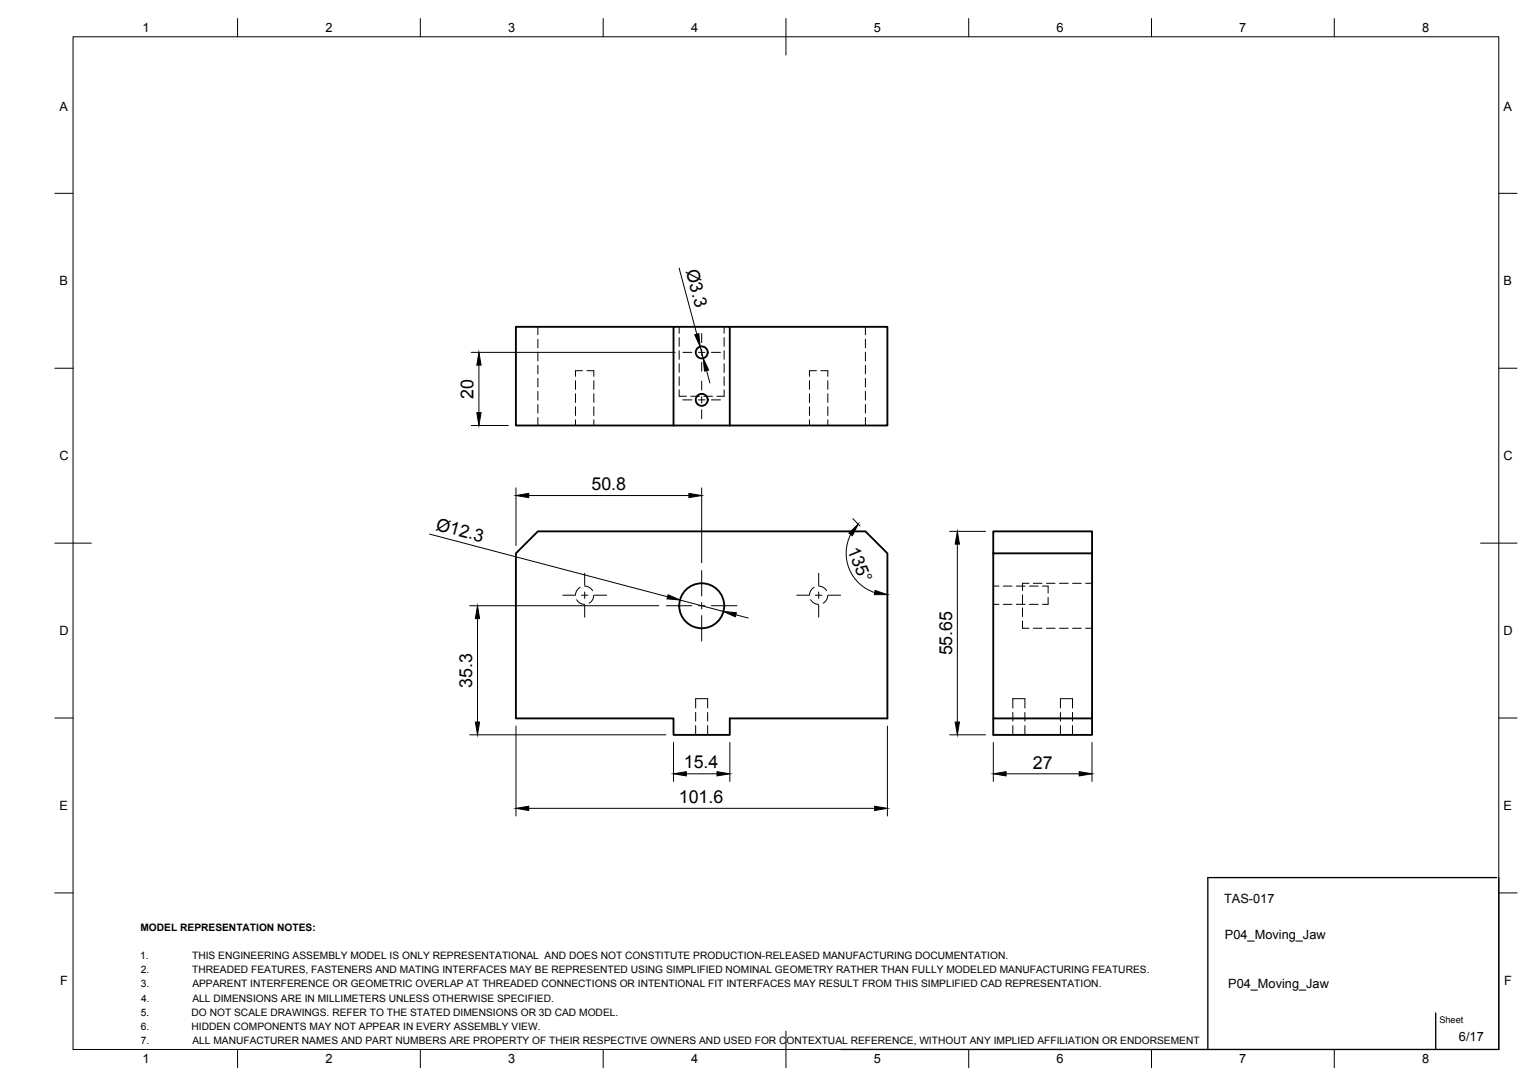
ISO-10303-21;
HEADER;
/* Generated by software containing ST-Developer
 * from STEP Tools, Inc. (www.steptools.com) 
 */

FILE_DESCRIPTION(
/* description */ ('STEP AP203'),
/* implementation_level */ '2;1');

FILE_NAME(
/* name */ 'P04_Moving_Jaw.step',
/* time_stamp */ '2026-11-15T15:04:01-08:00',
/* author */ (''),
/* organization */ (''),
/* preprocessor_version */ 'ST-DEVELOPER v20.2',
/* originating_system */ 'Autodesk Translation Framework v15.17.0.0',
/* authorisation */ '');

FILE_SCHEMA (('AUTOMOTIVE_DESIGN { 1 0 10303 214 3 1 1 }'));
ENDSEC;

DATA;
#10=MECHANICAL_DESIGN_GEOMETRIC_PRESENTATION_REPRESENTATION('',(#283,#284,#285),#16598);
#207=SHAPE_REPRESENTATION_RELATIONSHIP('SRR','None',#16701,#231);
#231=ADVANCED_BREP_SHAPE_REPRESENTATION('',(#255),#16577);
#255=MANIFOLD_SOLID_BREP('Body1',#9790);
#283=STYLED_ITEM('',(#16828),#9385);
#284=STYLED_ITEM('',(#16828),#9386);
#285=STYLED_ITEM('',(#16831),#255);
#331=FACE_BOUND('',#1644,.T.);
#332=FACE_BOUND('',#1645,.T.);
#333=FACE_BOUND('',#1647,.T.);
#334=FACE_BOUND('',#1651,.T.);
#335=FACE_BOUND('',#1652,.T.);
#558=PLANE('',#10282);
#559=PLANE('',#10283);
#560=PLANE('',#10284);
#561=PLANE('',#10285);
#562=PLANE('',#10286);
#563=PLANE('',#10287);
#564=PLANE('',#10288);
#565=PLANE('',#10289);
#566=PLANE('',#10290);
#567=PLANE('',#10291);
#568=PLANE('',#10292);
#569=PLANE('',#10293);
#570=PLANE('',#10294);
#571=PLANE('',#10295);
#572=PLANE('',#10296);
#573=PLANE('',#10297);
#574=PLANE('',#10298);
#1055=FACE_OUTER_BOUND('',#1631,.T.);
#1056=FACE_OUTER_BOUND('',#1632,.T.);
#1057=FACE_OUTER_BOUND('',#1633,.T.);
#1058=FACE_OUTER_BOUND('',#1634,.T.);
#1059=FACE_OUTER_BOUND('',#1635,.T.);
#1060=FACE_OUTER_BOUND('',#1636,.T.);
#1061=FACE_OUTER_BOUND('',#1637,.T.);
#1062=FACE_OUTER_BOUND('',#1638,.T.);
#1063=FACE_OUTER_BOUND('',#1639,.T.);
#1064=FACE_OUTER_BOUND('',#1640,.T.);
#1065=FACE_OUTER_BOUND('',#1641,.T.);
#1066=FACE_OUTER_BOUND('',#1642,.T.);
#1067=FACE_OUTER_BOUND('',#1643,.T.);
#1068=FACE_OUTER_BOUND('',#1646,.T.);
#1069=FACE_OUTER_BOUND('',#1648,.T.);
#1070=FACE_OUTER_BOUND('',#1649,.T.);
#1071=FACE_OUTER_BOUND('',#1650,.T.);
#1072=FACE_OUTER_BOUND('',#1653,.T.);
#1073=FACE_OUTER_BOUND('',#1654,.T.);
#1074=FACE_OUTER_BOUND('',#1655,.T.);
#1075=FACE_OUTER_BOUND('',#1656,.T.);
#1076=FACE_OUTER_BOUND('',#1657,.T.);
#1631=EDGE_LOOP('',(#7371,#7372,#7373,#7374));
#1632=EDGE_LOOP('',(#7375,#7376,#7377,#7378));
#1633=EDGE_LOOP('',(#7379,#7380,#7381,#7382));
#1634=EDGE_LOOP('',(#7383,#7384,#7385,#7386));
#1635=EDGE_LOOP('',(#7387,#7388,#7389,#7390));
#1636=EDGE_LOOP('',(#7391,#7392,#7393,#7394));
#1637=EDGE_LOOP('',(#7395,#7396,#7397,#7398));
#1638=EDGE_LOOP('',(#7399,#7400,#7401,#7402));
#1639=EDGE_LOOP('',(#7403,#7404,#7405,#7406));
#1640=EDGE_LOOP('',(#7407,#7408,#7409,#7410));
#1641=EDGE_LOOP('',(#7411,#7412,#7413,#7414));
#1642=EDGE_LOOP('',(#7415,#7416,#7417,#7418));
#1643=EDGE_LOOP('',(#7419,#7420,#7421,#7422,#7423,#7424,#7425,#7426,#7427,
#7428));
#1644=EDGE_LOOP('',(#7429));
#1645=EDGE_LOOP('',(#7430));
#1646=EDGE_LOOP('',(#7431,#7432,#7433,#7434,#7435,#7436,#7437,#7438,#7439,
#7440));
#1647=EDGE_LOOP('',(#7441));
#1648=EDGE_LOOP('',(#7442,#7443,#7444,#7445));
#1649=EDGE_LOOP('',(#7446,#7447,#7448,#7449));
#1650=EDGE_LOOP('',(#7450,#7451,#7452,#7453));
#1651=EDGE_LOOP('',(#7454));
#1652=EDGE_LOOP('',(#7455));
#1653=EDGE_LOOP('',(#7456));
#1654=EDGE_LOOP('',(#7457));
#1655=EDGE_LOOP('',(#7458));
#1656=EDGE_LOOP('',(#7459));
#1657=EDGE_LOOP('',(#7460));
#2481=LINE('',#14478,#3529);
#2482=LINE('',#14484,#3530);
#2483=LINE('',#14490,#3531);
#2484=LINE('',#14496,#3532);
#2485=LINE('',#14502,#3533);
#2486=LINE('',#14507,#3534);
#2487=LINE('',#14509,#3535);
#2488=LINE('',#14511,#3536);
#2489=LINE('',#14512,#3537);
#2490=LINE('',#14516,#3538);
#2491=LINE('',#14518,#3539);
#2492=LINE('',#14520,#3540);
#2493=LINE('',#14521,#3541);
#2494=LINE('',#14524,#3542);
#2495=LINE('',#14526,#3543);
#2496=LINE('',#14527,#3544);
#2497=LINE('',#14530,#3545);
#2498=LINE('',#14532,#3546);
#2499=LINE('',#14533,#3547);
#2500=LINE('',#14536,#3548);
#2501=LINE('',#14538,#3549);
#2502=LINE('',#14539,#3550);
#2503=LINE('',#14542,#3551);
#2504=LINE('',#14544,#3552);
#2505=LINE('',#14545,#3553);
#2506=LINE('',#14547,#3554);
#2507=LINE('',#14548,#3555);
#2508=LINE('',#14551,#3556);
#2509=LINE('',#14553,#3557);
#2510=LINE('',#14554,#3558);
#2511=LINE('',#14557,#3559);
#2512=LINE('',#14559,#3560);
#2513=LINE('',#14560,#3561);
#2514=LINE('',#14562,#3562);
#2515=LINE('',#14564,#3563);
#3529=VECTOR('',#11659,1.65);
#3530=VECTOR('',#11666,1.65);
#3531=VECTOR('',#11673,2.5);
#3532=VECTOR('',#11680,2.5);
#3533=VECTOR('',#11687,6.15);
#3534=VECTOR('',#11692,1000.);
#3535=VECTOR('',#11693,1000.);
#3536=VECTOR('',#11694,1000.);
#3537=VECTOR('',#11695,1000.);
#3538=VECTOR('',#11698,1000.);
#3539=VECTOR('',#11699,1000.);
#3540=VECTOR('',#11700,1000.);
#3541=VECTOR('',#11701,1000.);
#3542=VECTOR('',#11704,1000.);
#3543=VECTOR('',#11705,1000.);
#3544=VECTOR('',#11706,1000.);
#3545=VECTOR('',#11709,1000.);
#3546=VECTOR('',#11710,1000.);
#3547=VECTOR('',#11711,1000.);
#3548=VECTOR('',#11714,1000.);
#3549=VECTOR('',#11715,1000.);
#3550=VECTOR('',#11716,1000.);
#3551=VECTOR('',#11719,1000.);
#3552=VECTOR('',#11720,1000.);
#3553=VECTOR('',#11721,1000.);
#3554=VECTOR('',#11724,1000.);
#3555=VECTOR('',#11725,1000.);
#3556=VECTOR('',#11728,1000.);
#3557=VECTOR('',#11729,1000.);
#3558=VECTOR('',#11730,1000.);
#3559=VECTOR('',#11733,1000.);
#3560=VECTOR('',#11734,1000.);
#3561=VECTOR('',#11735,1000.);
#3562=VECTOR('',#11738,1000.);
#3563=VECTOR('',#11741,1000.);
#4265=CIRCLE('',#10268,1.65);
#4266=CIRCLE('',#10269,1.65);
#4267=CIRCLE('',#10271,1.65);
#4268=CIRCLE('',#10272,1.65);
#4269=CIRCLE('',#10274,2.5);
#4270=CIRCLE('',#10275,2.5);
#4271=CIRCLE('',#10277,2.5);
#4272=CIRCLE('',#10278,2.5);
#4273=CIRCLE('',#10280,6.15);
#4274=CIRCLE('',#10281,6.15);
#4713=VERTEX_POINT('',#14475);
#4714=VERTEX_POINT('',#14477);
#4715=VERTEX_POINT('',#14481);
#4716=VERTEX_POINT('',#14483);
#4717=VERTEX_POINT('',#14487);
#4718=VERTEX_POINT('',#14489);
#4719=VERTEX_POINT('',#14493);
#4720=VERTEX_POINT('',#14495);
#4721=VERTEX_POINT('',#14499);
#4722=VERTEX_POINT('',#14501);
#4723=VERTEX_POINT('',#14505);
#4724=VERTEX_POINT('',#14506);
#4725=VERTEX_POINT('',#14508);
#4726=VERTEX_POINT('',#14510);
#4727=VERTEX_POINT('',#14514);
#4728=VERTEX_POINT('',#14515);
#4729=VERTEX_POINT('',#14517);
#4730=VERTEX_POINT('',#14519);
#4731=VERTEX_POINT('',#14523);
#4732=VERTEX_POINT('',#14525);
#4733=VERTEX_POINT('',#14529);
#4734=VERTEX_POINT('',#14531);
#4735=VERTEX_POINT('',#14535);
#4736=VERTEX_POINT('',#14537);
#4737=VERTEX_POINT('',#14541);
#4738=VERTEX_POINT('',#14543);
#4739=VERTEX_POINT('',#14550);
#4740=VERTEX_POINT('',#14552);
#4741=VERTEX_POINT('',#14556);
#4742=VERTEX_POINT('',#14558);
#5698=EDGE_CURVE('',#4713,#4713,#4265,.T.);
#5699=EDGE_CURVE('',#4713,#4714,#2481,.T.);
#5700=EDGE_CURVE('',#4714,#4714,#4266,.T.);
#5701=EDGE_CURVE('',#4715,#4715,#4267,.T.);
#5702=EDGE_CURVE('',#4715,#4716,#2482,.T.);
#5703=EDGE_CURVE('',#4716,#4716,#4268,.T.);
#5704=EDGE_CURVE('',#4717,#4717,#4269,.T.);
#5705=EDGE_CURVE('',#4717,#4718,#2483,.T.);
#5706=EDGE_CURVE('',#4718,#4718,#4270,.T.);
#5707=EDGE_CURVE('',#4719,#4719,#4271,.T.);
#5708=EDGE_CURVE('',#4719,#4720,#2484,.T.);
#5709=EDGE_CURVE('',#4720,#4720,#4272,.T.);
#5710=EDGE_CURVE('',#4721,#4721,#4273,.T.);
#5711=EDGE_CURVE('',#4721,#4722,#2485,.T.);
#5712=EDGE_CURVE('',#4722,#4722,#4274,.T.);
#5713=EDGE_CURVE('',#4723,#4724,#2486,.T.);
#5714=EDGE_CURVE('',#4725,#4723,#2487,.T.);
#5715=EDGE_CURVE('',#4725,#4726,#2488,.T.);
#5716=EDGE_CURVE('',#4726,#4724,#2489,.T.);
#5717=EDGE_CURVE('',#4727,#4728,#2490,.T.);
#5718=EDGE_CURVE('',#4727,#4729,#2491,.T.);
#5719=EDGE_CURVE('',#4730,#4729,#2492,.T.);
#5720=EDGE_CURVE('',#4728,#4730,#2493,.T.);
#5721=EDGE_CURVE('',#4729,#4731,#2494,.T.);
#5722=EDGE_CURVE('',#4732,#4731,#2495,.T.);
#5723=EDGE_CURVE('',#4730,#4732,#2496,.T.);
#5724=EDGE_CURVE('',#4731,#4733,#2497,.T.);
#5725=EDGE_CURVE('',#4734,#4733,#2498,.T.);
#5726=EDGE_CURVE('',#4732,#4734,#2499,.T.);
#5727=EDGE_CURVE('',#4733,#4735,#2500,.T.);
#5728=EDGE_CURVE('',#4736,#4735,#2501,.T.);
#5729=EDGE_CURVE('',#4734,#4736,#2502,.T.);
#5730=EDGE_CURVE('',#4735,#4737,#2503,.T.);
#5731=EDGE_CURVE('',#4738,#4737,#2504,.T.);
#5732=EDGE_CURVE('',#4736,#4738,#2505,.T.);
#5733=EDGE_CURVE('',#4737,#4726,#2506,.T.);
#5734=EDGE_CURVE('',#4738,#4725,#2507,.T.);
#5735=EDGE_CURVE('',#4723,#4739,#2508,.T.);
#5736=EDGE_CURVE('',#4739,#4740,#2509,.T.);
#5737=EDGE_CURVE('',#4728,#4740,#2510,.T.);
#5738=EDGE_CURVE('',#4727,#4741,#2511,.T.);
#5739=EDGE_CURVE('',#4741,#4742,#2512,.T.);
#5740=EDGE_CURVE('',#4724,#4742,#2513,.T.);
#5741=EDGE_CURVE('',#4742,#4739,#2514,.T.);
#5742=EDGE_CURVE('',#4740,#4741,#2515,.T.);
#7371=ORIENTED_EDGE('',*,*,#5698,.T.);
#7372=ORIENTED_EDGE('',*,*,#5699,.T.);
#7373=ORIENTED_EDGE('',*,*,#5700,.F.);
#7374=ORIENTED_EDGE('',*,*,#5699,.F.);
#7375=ORIENTED_EDGE('',*,*,#5701,.T.);
#7376=ORIENTED_EDGE('',*,*,#5702,.T.);
#7377=ORIENTED_EDGE('',*,*,#5703,.F.);
#7378=ORIENTED_EDGE('',*,*,#5702,.F.);
#7379=ORIENTED_EDGE('',*,*,#5704,.T.);
#7380=ORIENTED_EDGE('',*,*,#5705,.T.);
#7381=ORIENTED_EDGE('',*,*,#5706,.F.);
#7382=ORIENTED_EDGE('',*,*,#5705,.F.);
#7383=ORIENTED_EDGE('',*,*,#5707,.T.);
#7384=ORIENTED_EDGE('',*,*,#5708,.T.);
#7385=ORIENTED_EDGE('',*,*,#5709,.F.);
#7386=ORIENTED_EDGE('',*,*,#5708,.F.);
#7387=ORIENTED_EDGE('',*,*,#5710,.T.);
#7388=ORIENTED_EDGE('',*,*,#5711,.T.);
#7389=ORIENTED_EDGE('',*,*,#5712,.F.);
#7390=ORIENTED_EDGE('',*,*,#5711,.F.);
#7391=ORIENTED_EDGE('',*,*,#5713,.F.);
#7392=ORIENTED_EDGE('',*,*,#5714,.F.);
#7393=ORIENTED_EDGE('',*,*,#5715,.T.);
#7394=ORIENTED_EDGE('',*,*,#5716,.T.);
#7395=ORIENTED_EDGE('',*,*,#5717,.F.);
#7396=ORIENTED_EDGE('',*,*,#5718,.T.);
#7397=ORIENTED_EDGE('',*,*,#5719,.F.);
#7398=ORIENTED_EDGE('',*,*,#5720,.F.);
#7399=ORIENTED_EDGE('',*,*,#5721,.T.);
#7400=ORIENTED_EDGE('',*,*,#5722,.F.);
#7401=ORIENTED_EDGE('',*,*,#5723,.F.);
#7402=ORIENTED_EDGE('',*,*,#5719,.T.);
#7403=ORIENTED_EDGE('',*,*,#5724,.T.);
#7404=ORIENTED_EDGE('',*,*,#5725,.F.);
#7405=ORIENTED_EDGE('',*,*,#5726,.F.);
#7406=ORIENTED_EDGE('',*,*,#5722,.T.);
#7407=ORIENTED_EDGE('',*,*,#5727,.T.);
#7408=ORIENTED_EDGE('',*,*,#5728,.F.);
#7409=ORIENTED_EDGE('',*,*,#5729,.F.);
#7410=ORIENTED_EDGE('',*,*,#5725,.T.);
#7411=ORIENTED_EDGE('',*,*,#5730,.T.);
#7412=ORIENTED_EDGE('',*,*,#5731,.F.);
#7413=ORIENTED_EDGE('',*,*,#5732,.F.);
#7414=ORIENTED_EDGE('',*,*,#5728,.T.);
#7415=ORIENTED_EDGE('',*,*,#5733,.T.);
#7416=ORIENTED_EDGE('',*,*,#5715,.F.);
#7417=ORIENTED_EDGE('',*,*,#5734,.F.);
#7418=ORIENTED_EDGE('',*,*,#5731,.T.);
#7419=ORIENTED_EDGE('',*,*,#5714,.T.);
#7420=ORIENTED_EDGE('',*,*,#5735,.T.);
#7421=ORIENTED_EDGE('',*,*,#5736,.T.);
#7422=ORIENTED_EDGE('',*,*,#5737,.F.);
#7423=ORIENTED_EDGE('',*,*,#5720,.T.);
#7424=ORIENTED_EDGE('',*,*,#5723,.T.);
#7425=ORIENTED_EDGE('',*,*,#5726,.T.);
#7426=ORIENTED_EDGE('',*,*,#5729,.T.);
#7427=ORIENTED_EDGE('',*,*,#5732,.T.);
#7428=ORIENTED_EDGE('',*,*,#5734,.T.);
#7429=ORIENTED_EDGE('',*,*,#5704,.F.);
#7430=ORIENTED_EDGE('',*,*,#5707,.F.);
#7431=ORIENTED_EDGE('',*,*,#5718,.F.);
#7432=ORIENTED_EDGE('',*,*,#5738,.T.);
#7433=ORIENTED_EDGE('',*,*,#5739,.T.);
#7434=ORIENTED_EDGE('',*,*,#5740,.F.);
#7435=ORIENTED_EDGE('',*,*,#5716,.F.);
#7436=ORIENTED_EDGE('',*,*,#5733,.F.);
#7437=ORIENTED_EDGE('',*,*,#5730,.F.);
#7438=ORIENTED_EDGE('',*,*,#5727,.F.);
#7439=ORIENTED_EDGE('',*,*,#5724,.F.);
#7440=ORIENTED_EDGE('',*,*,#5721,.F.);
#7441=ORIENTED_EDGE('',*,*,#5712,.T.);
#7442=ORIENTED_EDGE('',*,*,#5735,.F.);
#7443=ORIENTED_EDGE('',*,*,#5713,.T.);
#7444=ORIENTED_EDGE('',*,*,#5740,.T.);
#7445=ORIENTED_EDGE('',*,*,#5741,.T.);
#7446=ORIENTED_EDGE('',*,*,#5738,.F.);
#7447=ORIENTED_EDGE('',*,*,#5717,.T.);
#7448=ORIENTED_EDGE('',*,*,#5737,.T.);
#7449=ORIENTED_EDGE('',*,*,#5742,.T.);
#7450=ORIENTED_EDGE('',*,*,#5741,.F.);
#7451=ORIENTED_EDGE('',*,*,#5739,.F.);
#7452=ORIENTED_EDGE('',*,*,#5742,.F.);
#7453=ORIENTED_EDGE('',*,*,#5736,.F.);
#7454=ORIENTED_EDGE('',*,*,#5700,.T.);
#7455=ORIENTED_EDGE('',*,*,#5703,.T.);
#7456=ORIENTED_EDGE('',*,*,#5710,.F.);
#7457=ORIENTED_EDGE('',*,*,#5709,.T.);
#7458=ORIENTED_EDGE('',*,*,#5706,.T.);
#7459=ORIENTED_EDGE('',*,*,#5701,.F.);
#7460=ORIENTED_EDGE('',*,*,#5698,.F.);
#9184=CYLINDRICAL_SURFACE('',#10267,1.65);
#9185=CYLINDRICAL_SURFACE('',#10270,1.65);
#9186=CYLINDRICAL_SURFACE('',#10273,2.5);
#9187=CYLINDRICAL_SURFACE('',#10276,2.5);
#9188=CYLINDRICAL_SURFACE('',#10279,6.15);
#9380=ADVANCED_FACE('',(#1055),#9184,.F.);
#9381=ADVANCED_FACE('',(#1056),#9185,.F.);
#9382=ADVANCED_FACE('',(#1057),#9186,.F.);
#9383=ADVANCED_FACE('',(#1058),#9187,.F.);
#9384=ADVANCED_FACE('',(#1059),#9188,.F.);
#9385=ADVANCED_FACE('',(#1060),#558,.F.);
#9386=ADVANCED_FACE('',(#1061),#559,.F.);
#9387=ADVANCED_FACE('',(#1062),#560,.F.);
#9388=ADVANCED_FACE('',(#1063),#561,.F.);
#9389=ADVANCED_FACE('',(#1064),#562,.F.);
#9390=ADVANCED_FACE('',(#1065),#563,.F.);
#9391=ADVANCED_FACE('',(#1066),#564,.F.);
#9392=ADVANCED_FACE('',(#1067,#331,#332),#565,.F.);
#9393=ADVANCED_FACE('',(#1068,#333),#566,.T.);
#9394=ADVANCED_FACE('',(#1069),#567,.F.);
#9395=ADVANCED_FACE('',(#1070),#568,.F.);
#9396=ADVANCED_FACE('',(#1071,#334,#335),#569,.T.);
#9397=ADVANCED_FACE('',(#1072),#570,.F.);
#9398=ADVANCED_FACE('',(#1073),#571,.T.);
#9399=ADVANCED_FACE('',(#1074),#572,.T.);
#9400=ADVANCED_FACE('',(#1075),#573,.F.);
#9401=ADVANCED_FACE('',(#1076),#574,.F.);
#9790=CLOSED_SHELL('',(#9380,#9381,#9382,#9383,#9384,#9385,#9386,#9387,
#9388,#9389,#9390,#9391,#9392,#9393,#9394,#9395,#9396,#9397,#9398,#9399,
#9400,#9401));
#10266=AXIS2_PLACEMENT_3D('',#14473,#11653,#11654);
#10267=AXIS2_PLACEMENT_3D('',#14474,#11655,#11656);
#10268=AXIS2_PLACEMENT_3D('',#14476,#11657,#11658);
#10269=AXIS2_PLACEMENT_3D('',#14479,#11660,#11661);
#10270=AXIS2_PLACEMENT_3D('',#14480,#11662,#11663);
#10271=AXIS2_PLACEMENT_3D('',#14482,#11664,#11665);
#10272=AXIS2_PLACEMENT_3D('',#14485,#11667,#11668);
#10273=AXIS2_PLACEMENT_3D('',#14486,#11669,#11670);
#10274=AXIS2_PLACEMENT_3D('',#14488,#11671,#11672);
#10275=AXIS2_PLACEMENT_3D('',#14491,#11674,#11675);
#10276=AXIS2_PLACEMENT_3D('',#14492,#11676,#11677);
#10277=AXIS2_PLACEMENT_3D('',#14494,#11678,#11679);
#10278=AXIS2_PLACEMENT_3D('',#14497,#11681,#11682);
#10279=AXIS2_PLACEMENT_3D('',#14498,#11683,#11684);
#10280=AXIS2_PLACEMENT_3D('',#14500,#11685,#11686);
#10281=AXIS2_PLACEMENT_3D('',#14503,#11688,#11689);
#10282=AXIS2_PLACEMENT_3D('',#14504,#11690,#11691);
#10283=AXIS2_PLACEMENT_3D('',#14513,#11696,#11697);
#10284=AXIS2_PLACEMENT_3D('',#14522,#11702,#11703);
#10285=AXIS2_PLACEMENT_3D('',#14528,#11707,#11708);
#10286=AXIS2_PLACEMENT_3D('',#14534,#11712,#11713);
#10287=AXIS2_PLACEMENT_3D('',#14540,#11717,#11718);
#10288=AXIS2_PLACEMENT_3D('',#14546,#11722,#11723);
#10289=AXIS2_PLACEMENT_3D('',#14549,#11726,#11727);
#10290=AXIS2_PLACEMENT_3D('',#14555,#11731,#11732);
#10291=AXIS2_PLACEMENT_3D('',#14561,#11736,#11737);
#10292=AXIS2_PLACEMENT_3D('',#14563,#11739,#11740);
#10293=AXIS2_PLACEMENT_3D('',#14565,#11742,#11743);
#10294=AXIS2_PLACEMENT_3D('',#14566,#11744,#11745);
#10295=AXIS2_PLACEMENT_3D('',#14567,#11746,#11747);
#10296=AXIS2_PLACEMENT_3D('',#14568,#11748,#11749);
#10297=AXIS2_PLACEMENT_3D('',#14569,#11750,#11751);
#10298=AXIS2_PLACEMENT_3D('',#14570,#11752,#11753);
#11653=DIRECTION('axis',(0.,0.,1.));
#11654=DIRECTION('refdir',(1.,0.,0.));
#11655=DIRECTION('center_axis',(0.,0.,-1.));
#11656=DIRECTION('ref_axis',(-1.,0.,0.));
#11657=DIRECTION('center_axis',(0.,0.,1.));
#11658=DIRECTION('ref_axis',(1.,0.,0.));
#11659=DIRECTION('',(0.,0.,-1.));
#11660=DIRECTION('center_axis',(0.,0.,1.));
#11661=DIRECTION('ref_axis',(-1.,0.,0.));
#11662=DIRECTION('center_axis',(0.,0.,-1.));
#11663=DIRECTION('ref_axis',(-1.,0.,0.));
#11664=DIRECTION('center_axis',(0.,0.,1.));
#11665=DIRECTION('ref_axis',(1.,0.,0.));
#11666=DIRECTION('',(0.,0.,-1.));
#11667=DIRECTION('center_axis',(0.,0.,1.));
#11668=DIRECTION('ref_axis',(-1.,0.,0.));
#11669=DIRECTION('center_axis',(0.,-1.,0.));
#11670=DIRECTION('ref_axis',(0.,0.,-1.));
#11671=DIRECTION('center_axis',(0.,1.,0.));
#11672=DIRECTION('ref_axis',(0.,0.,-1.));
#11673=DIRECTION('',(0.,-1.,0.));
#11674=DIRECTION('center_axis',(0.,1.,0.));
#11675=DIRECTION('ref_axis',(0.,0.,1.));
#11676=DIRECTION('center_axis',(0.,-1.,0.));
#11677=DIRECTION('ref_axis',(0.,0.,-1.));
#11678=DIRECTION('center_axis',(0.,1.,0.));
#11679=DIRECTION('ref_axis',(0.,0.,-1.));
#11680=DIRECTION('',(0.,-1.,0.));
#11681=DIRECTION('center_axis',(0.,1.,0.));
#11682=DIRECTION('ref_axis',(0.,0.,1.));
#11683=DIRECTION('center_axis',(0.,-1.,0.));
#11684=DIRECTION('ref_axis',(0.,0.,-1.));
#11685=DIRECTION('center_axis',(0.,1.,0.));
#11686=DIRECTION('ref_axis',(0.,0.,1.));
#11687=DIRECTION('',(0.,-1.,0.));
#11688=DIRECTION('center_axis',(0.,1.,0.));
#11689=DIRECTION('ref_axis',(0.,0.,-1.));
#11690=DIRECTION('center_axis',(0.,0.,1.));
#11691=DIRECTION('ref_axis',(1.,0.,0.));
#11692=DIRECTION('',(0.,-1.,0.));
#11693=DIRECTION('',(-1.,0.,0.));
#11694=DIRECTION('',(0.,-1.,0.));
#11695=DIRECTION('',(-1.,0.,0.));
#11696=DIRECTION('center_axis',(0.,0.,1.));
#11697=DIRECTION('ref_axis',(1.,0.,0.));
#11698=DIRECTION('',(0.,1.,0.));
#11699=DIRECTION('',(-1.,0.,0.));
#11700=DIRECTION('',(0.,-1.,0.));
#11701=DIRECTION('',(-1.,0.,0.));
#11702=DIRECTION('center_axis',(1.,0.,0.));
#11703=DIRECTION('ref_axis',(0.,0.,-1.));
#11704=DIRECTION('',(0.,0.,1.));
#11705=DIRECTION('',(0.,-1.,0.));
#11706=DIRECTION('',(0.,0.,1.));
#11707=DIRECTION('center_axis',(0.70710678118654,0.,-0.707106781186555));
#11708=DIRECTION('ref_axis',(-0.707106781186555,0.,-0.70710678118654));
#11709=DIRECTION('',(0.707106781186555,0.,0.70710678118654));
#11710=DIRECTION('',(0.,-1.,0.));
#11711=DIRECTION('',(0.707106781186555,0.,0.70710678118654));
#11712=DIRECTION('center_axis',(0.,0.,-1.));
#11713=DIRECTION('ref_axis',(-1.,0.,0.));
#11714=DIRECTION('',(1.,0.,0.));
#11715=DIRECTION('',(0.,-1.,0.));
#11716=DIRECTION('',(1.,0.,0.));
#11717=DIRECTION('center_axis',(-0.707106781186565,0.,-0.70710678118653));
#11718=DIRECTION('ref_axis',(-0.70710678118653,0.,0.707106781186565));
#11719=DIRECTION('',(0.70710678118653,0.,-0.707106781186565));
#11720=DIRECTION('',(0.,-1.,0.));
#11721=DIRECTION('',(0.70710678118653,0.,-0.707106781186565));
#11722=DIRECTION('center_axis',(-1.,0.,0.));
#11723=DIRECTION('ref_axis',(0.,0.,1.));
#11724=DIRECTION('',(0.,0.,-1.));
#11725=DIRECTION('',(0.,0.,-1.));
#11726=DIRECTION('center_axis',(0.,-1.,0.));
#11727=DIRECTION('ref_axis',(0.,0.,-1.));
#11728=DIRECTION('',(0.,0.,-1.));
#11729=DIRECTION('',(-1.,0.,0.));
#11730=DIRECTION('',(0.,0.,-1.));
#11731=DIRECTION('center_axis',(0.,-1.,0.));
#11732=DIRECTION('ref_axis',(0.,0.,-1.));
#11733=DIRECTION('',(0.,0.,-1.));
#11734=DIRECTION('',(1.,0.,0.));
#11735=DIRECTION('',(0.,0.,-1.));
#11736=DIRECTION('center_axis',(-1.,0.,0.));
#11737=DIRECTION('ref_axis',(0.,0.,1.));
#11738=DIRECTION('',(0.,1.,0.));
#11739=DIRECTION('center_axis',(1.,0.,0.));
#11740=DIRECTION('ref_axis',(0.,0.,-1.));
#11741=DIRECTION('',(0.,-1.,0.));
#11742=DIRECTION('center_axis',(0.,0.,-1.));
#11743=DIRECTION('ref_axis',(-1.,0.,0.));
#11744=DIRECTION('center_axis',(0.,1.,0.));
#11745=DIRECTION('ref_axis',(0.,0.,1.));
#11746=DIRECTION('center_axis',(0.,1.,0.));
#11747=DIRECTION('ref_axis',(0.,0.,1.));
#11748=DIRECTION('center_axis',(0.,1.,0.));
#11749=DIRECTION('ref_axis',(0.,0.,1.));
#11750=DIRECTION('center_axis',(0.,0.,1.));
#11751=DIRECTION('ref_axis',(1.,0.,0.));
#11752=DIRECTION('center_axis',(0.,0.,1.));
#11753=DIRECTION('ref_axis',(1.,0.,0.));
#14473=CARTESIAN_POINT('',(0.,0.,0.));
#14474=CARTESIAN_POINT('Origin',(0.,5.,87.6));
#14475=CARTESIAN_POINT('',(1.65,5.,87.6));
#14476=CARTESIAN_POINT('Origin',(0.,5.,87.6));
#14477=CARTESIAN_POINT('',(1.65,5.,77.7));
#14478=CARTESIAN_POINT('',(1.65,5.,87.6));
#14479=CARTESIAN_POINT('Origin',(0.,5.,77.7));
#14480=CARTESIAN_POINT('Origin',(0.,18.,87.6));
#14481=CARTESIAN_POINT('',(1.65,18.,87.6));
#14482=CARTESIAN_POINT('Origin',(0.,18.,87.6));
#14483=CARTESIAN_POINT('',(1.65,18.,77.7));
#14484=CARTESIAN_POINT('',(1.65,18.,87.6));
#14485=CARTESIAN_POINT('Origin',(0.,18.,77.7));
#14486=CARTESIAN_POINT('Origin',(-32.,26.,115.8875));
#14487=CARTESIAN_POINT('',(-32.,25.,118.3875));
#14488=CARTESIAN_POINT('Origin',(-32.,25.,115.8875));
#14489=CARTESIAN_POINT('',(-32.,10.,118.3875));
#14490=CARTESIAN_POINT('',(-32.,26.,118.3875));
#14491=CARTESIAN_POINT('Origin',(-32.,10.,115.8875));
#14492=CARTESIAN_POINT('Origin',(32.,26.,115.8875));
#14493=CARTESIAN_POINT('',(32.,25.,118.3875));
#14494=CARTESIAN_POINT('Origin',(32.,25.,115.8875));
#14495=CARTESIAN_POINT('',(32.,10.,118.3875));
#14496=CARTESIAN_POINT('',(32.,26.,118.3875));
#14497=CARTESIAN_POINT('Origin',(32.,10.,115.8875));
#14498=CARTESIAN_POINT('Origin',(0.,17.,113.));
#14499=CARTESIAN_POINT('',(-7.53157781475623E-16,17.,119.15));
#14500=CARTESIAN_POINT('Origin',(0.,17.,113.));
#14501=CARTESIAN_POINT('',(-7.53157781475623E-16,-2.,119.15));
#14502=CARTESIAN_POINT('',(-7.53157781475623E-16,17.,119.15));
#14503=CARTESIAN_POINT('Origin',(0.,-2.,113.));
#14504=CARTESIAN_POINT('Origin',(-50.8,25.,82.2));
#14505=CARTESIAN_POINT('',(7.7,25.,82.2));
#14506=CARTESIAN_POINT('',(7.7,-2.,82.2));
#14507=CARTESIAN_POINT('',(7.7,25.,82.2));
#14508=CARTESIAN_POINT('',(50.8,25.,82.2));
#14509=CARTESIAN_POINT('',(-50.8,25.,82.2));
#14510=CARTESIAN_POINT('',(50.8,-2.,82.2));
#14511=CARTESIAN_POINT('',(50.8,25.,82.2));
#14512=CARTESIAN_POINT('',(-50.8,-2.,82.2));
#14513=CARTESIAN_POINT('Origin',(-50.8,25.,82.2));
#14514=CARTESIAN_POINT('',(-7.7,-2.,82.2));
#14515=CARTESIAN_POINT('',(-7.7,25.,82.2));
#14516=CARTESIAN_POINT('',(-7.7,25.,82.2));
#14517=CARTESIAN_POINT('',(-50.8,-2.,82.2));
#14518=CARTESIAN_POINT('',(-50.8,-2.,82.2));
#14519=CARTESIAN_POINT('',(-50.8,25.,82.2));
#14520=CARTESIAN_POINT('',(-50.8,25.,82.2));
#14521=CARTESIAN_POINT('',(-50.8,25.,82.2));
#14522=CARTESIAN_POINT('Origin',(-50.8,25.,127.35));
#14523=CARTESIAN_POINT('',(-50.8,-2.,127.35));
#14524=CARTESIAN_POINT('',(-50.8,-2.,127.35));
#14525=CARTESIAN_POINT('',(-50.8,25.,127.35));
#14526=CARTESIAN_POINT('',(-50.8,25.,127.35));
#14527=CARTESIAN_POINT('',(-50.8,25.,127.35));
#14528=CARTESIAN_POINT('Origin',(-44.8,25.,133.35));
#14529=CARTESIAN_POINT('',(-44.8,-2.,133.35));
#14530=CARTESIAN_POINT('',(-44.8,-2.,133.35));
#14531=CARTESIAN_POINT('',(-44.8,25.,133.35));
#14532=CARTESIAN_POINT('',(-44.8,25.,133.35));
#14533=CARTESIAN_POINT('',(-44.8,25.,133.35));
#14534=CARTESIAN_POINT('Origin',(44.8000000000001,25.,133.35));
#14535=CARTESIAN_POINT('',(44.8000000000001,-2.,133.35));
#14536=CARTESIAN_POINT('',(44.8000000000001,-2.,133.35));
#14537=CARTESIAN_POINT('',(44.8000000000001,25.,133.35));
#14538=CARTESIAN_POINT('',(44.8000000000001,25.,133.35));
#14539=CARTESIAN_POINT('',(44.8000000000001,25.,133.35));
#14540=CARTESIAN_POINT('Origin',(50.8,25.,127.35));
#14541=CARTESIAN_POINT('',(50.8,-2.,127.35));
#14542=CARTESIAN_POINT('',(50.8,-2.,127.35));
#14543=CARTESIAN_POINT('',(50.8,25.,127.35));
#14544=CARTESIAN_POINT('',(50.8,25.,127.35));
#14545=CARTESIAN_POINT('',(50.8,25.,127.35));
#14546=CARTESIAN_POINT('Origin',(50.8,25.,82.2));
#14547=CARTESIAN_POINT('',(50.8,-2.,82.2));
#14548=CARTESIAN_POINT('',(50.8,25.,82.2));
#14549=CARTESIAN_POINT('Origin',(0.,25.,0.));
#14550=CARTESIAN_POINT('',(7.7,25.,77.7));
#14551=CARTESIAN_POINT('',(7.7,25.,84.2));
#14552=CARTESIAN_POINT('',(-7.7,25.,77.7));
#14553=CARTESIAN_POINT('',(-7.7,25.,77.7));
#14554=CARTESIAN_POINT('',(-7.7,25.,84.2));
#14555=CARTESIAN_POINT('Origin',(0.,-2.,0.));
#14556=CARTESIAN_POINT('',(-7.7,-2.,77.7));
#14557=CARTESIAN_POINT('',(-7.7,-2.,84.2));
#14558=CARTESIAN_POINT('',(7.7,-2.,77.7));
#14559=CARTESIAN_POINT('',(-7.7,-2.,77.7));
#14560=CARTESIAN_POINT('',(7.7,-2.,84.2));
#14561=CARTESIAN_POINT('Origin',(7.7,-2.,84.2));
#14562=CARTESIAN_POINT('',(7.7,-2.,77.7));
#14563=CARTESIAN_POINT('Origin',(-7.7,-2.,84.2));
#14564=CARTESIAN_POINT('',(-7.7,-2.,77.7));
#14565=CARTESIAN_POINT('Origin',(0.,0.,77.7));
#14566=CARTESIAN_POINT('Origin',(0.,17.,113.));
#14567=CARTESIAN_POINT('Origin',(32.,10.,115.8875));
#14568=CARTESIAN_POINT('Origin',(-32.,10.,115.8875));
#14569=CARTESIAN_POINT('Origin',(0.,18.,87.6));
#14570=CARTESIAN_POINT('Origin',(0.,5.,87.6));
#16551=UNCERTAINTY_MEASURE_WITH_UNIT(LENGTH_MEASURE(0.01),#16599,
'DISTANCE_ACCURACY_VALUE',
'Maximum model space distance between geometric entities at asserted c
onnectivities');
#16572=UNCERTAINTY_MEASURE_WITH_UNIT(LENGTH_MEASURE(0.01),#16599,
'DISTANCE_ACCURACY_VALUE',
'Maximum model space distance between geometric entities at asserted c
onnectivities');
#16577=(
GEOMETRIC_REPRESENTATION_CONTEXT(3)
GLOBAL_UNCERTAINTY_ASSIGNED_CONTEXT((#16551))
GLOBAL_UNIT_ASSIGNED_CONTEXT((#16599,#16601,#16602))
REPRESENTATION_CONTEXT('','3D')
);
#16598=(
GEOMETRIC_REPRESENTATION_CONTEXT(3)
GLOBAL_UNCERTAINTY_ASSIGNED_CONTEXT((#16572))
GLOBAL_UNIT_ASSIGNED_CONTEXT((#16599,#16601,#16602))
REPRESENTATION_CONTEXT('','3D')
);
#16599=(
LENGTH_UNIT()
NAMED_UNIT(*)
SI_UNIT(.MILLI.,.METRE.)
);
#16601=(
NAMED_UNIT(*)
PLANE_ANGLE_UNIT()
SI_UNIT($,.RADIAN.)
);
#16602=(
NAMED_UNIT(*)
SI_UNIT($,.STERADIAN.)
SOLID_ANGLE_UNIT()
);
#16607=SHAPE_DEFINITION_REPRESENTATION(#16632,#16701);
#16632=PRODUCT_DEFINITION_SHAPE('',$,#16727);
#16701=SHAPE_REPRESENTATION('',(#10266),#16577);
#16722=PRODUCT_DEFINITION_CONTEXT('part definition',#16799,'design');
#16727=PRODUCT_DEFINITION('P04_Moving_Jaw','P04_Moving_Jaw',#16752,#16722);
#16752=PRODUCT_DEFINITION_FORMATION('',$,#16805);
#16799=APPLICATION_CONTEXT(
'Core Data for Automotive Mechanical Design Process');
#16800=PRODUCT_CONTEXT('part definition',#16799,'mechanical');
#16805=PRODUCT('P04_Moving_Jaw','P04_Moving_Jaw',$,(#16800));
#16828=PRESENTATION_STYLE_ASSIGNMENT((#16837));
#16831=PRESENTATION_STYLE_ASSIGNMENT((#16840));
#16837=SURFACE_STYLE_USAGE(.BOTH.,#16846);
#16840=SURFACE_STYLE_USAGE(.BOTH.,#16849);
#16846=SURFACE_SIDE_STYLE('',(#16855));
#16849=SURFACE_SIDE_STYLE('',(#16858));
#16855=SURFACE_STYLE_FILL_AREA(#16864);
#16858=SURFACE_STYLE_FILL_AREA(#16867);
#16864=FILL_AREA_STYLE('Opaque(147,158,163)',(#16873));
#16867=FILL_AREA_STYLE('Black',(#16876));
#16873=FILL_AREA_STYLE_COLOUR('Opaque(147,158,163)',#16882);
#16876=FILL_AREA_STYLE_COLOUR('Black',#16885);
#16882=COLOUR_RGB('Opaque(147,158,163)',0.576470588235294,0.619607843137255,
0.63921568627451);
#16885=COLOUR_RGB('Black',0.0784313725490196,0.0784313725490196,0.0784313725490196);
ENDSEC;
END-ISO-10303-21;
